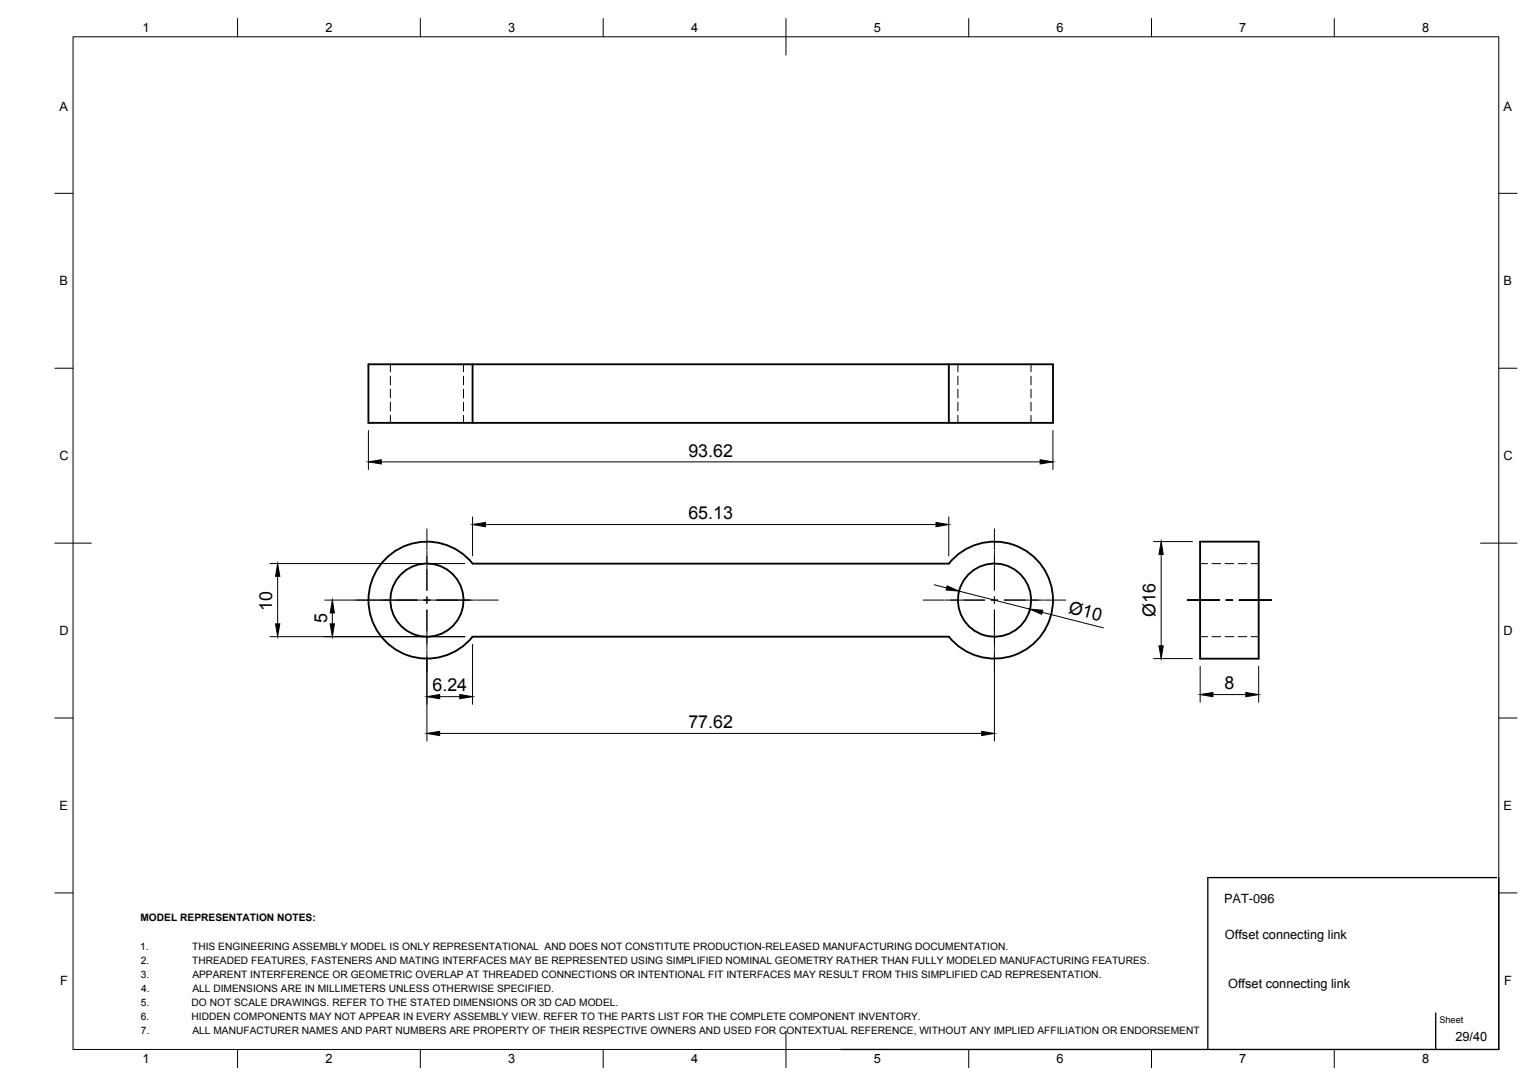
ISO-10303-21;
HEADER;
/* Generated by software containing ST-Developer
 * from STEP Tools, Inc. (www.steptools.com) 
 */

FILE_DESCRIPTION(
/* description */ ('PAT-096'),
/* implementation_level */ '2;1');

FILE_NAME(
/* name */ 'Offset connecting link.step',
/* time_stamp */ '2026-10-29T17:03:14-07:00',
/* author */ (''),
/* organization */ (''),
/* preprocessor_version */ 'ST-DEVELOPER v20.2',
/* originating_system */ 'Autodesk Translation Framework v15.17.0.0',
/* authorisation */ '');

FILE_SCHEMA (('AUTOMOTIVE_DESIGN { 1 0 10303 214 3 1 1 }'));
ENDSEC;

DATA;
#10=MECHANICAL_DESIGN_GEOMETRIC_PRESENTATION_REPRESENTATION('',(#426),#10650);
#356=SHAPE_REPRESENTATION_RELATIONSHIP('SRR','None',#10819,#387);
#387=ADVANCED_BREP_SHAPE_REPRESENTATION('',(#463),#10637);
#426=STYLED_ITEM('',(#11078),#463);
#463=MANIFOLD_SOLID_BREP('Body1',#5561);
#564=FACE_BOUND('',#1460,.T.);
#565=FACE_BOUND('',#1461,.T.);
#566=FACE_BOUND('',#1465,.T.);
#567=FACE_BOUND('',#1466,.T.);
#732=PLANE('',#6429);
#733=PLANE('',#6430);
#734=PLANE('',#6432);
#735=PLANE('',#6435);
#1028=FACE_OUTER_BOUND('',#1455,.T.);
#1029=FACE_OUTER_BOUND('',#1456,.T.);
#1030=FACE_OUTER_BOUND('',#1457,.T.);
#1031=FACE_OUTER_BOUND('',#1458,.T.);
#1032=FACE_OUTER_BOUND('',#1459,.T.);
#1033=FACE_OUTER_BOUND('',#1462,.T.);
#1034=FACE_OUTER_BOUND('',#1463,.T.);
#1035=FACE_OUTER_BOUND('',#1464,.T.);
#1455=EDGE_LOOP('',(#4695,#4696,#4697,#4698));
#1456=EDGE_LOOP('',(#4699,#4700,#4701,#4702));
#1457=EDGE_LOOP('',(#4703,#4704,#4705,#4706));
#1458=EDGE_LOOP('',(#4707,#4708,#4709,#4710));
#1459=EDGE_LOOP('',(#4711,#4712,#4713,#4714));
#1460=EDGE_LOOP('',(#4715));
#1461=EDGE_LOOP('',(#4716));
#1462=EDGE_LOOP('',(#4717,#4718,#4719,#4720));
#1463=EDGE_LOOP('',(#4721,#4722,#4723,#4724));
#1464=EDGE_LOOP('',(#4725,#4726,#4727,#4728));
#1465=EDGE_LOOP('',(#4729));
#1466=EDGE_LOOP('',(#4730));
#1824=LINE('',#10095,#2153);
#1825=LINE('',#10101,#2154);
#1826=LINE('',#10106,#2155);
#1827=LINE('',#10110,#2156);
#1828=LINE('',#10114,#2157);
#1829=LINE('',#10116,#2158);
#1830=LINE('',#10117,#2159);
#1831=LINE('',#10120,#2160);
#1832=LINE('',#10124,#2161);
#1833=LINE('',#10125,#2162);
#2153=VECTOR('',#7908,0.5);
#2154=VECTOR('',#7915,0.5);
#2155=VECTOR('',#7920,1.);
#2156=VECTOR('',#7923,1.);
#2157=VECTOR('',#7928,1.);
#2158=VECTOR('',#7929,1.);
#2159=VECTOR('',#7930,1.);
#2160=VECTOR('',#7933,1.);
#2161=VECTOR('',#7938,1.);
#2162=VECTOR('',#7939,1.);
#2495=CIRCLE('',#6421,0.5);
#2496=CIRCLE('',#6422,0.5);
#2497=CIRCLE('',#6424,0.5);
#2498=CIRCLE('',#6425,0.5);
#2499=CIRCLE('',#6427,0.800000000000001);
#2500=CIRCLE('',#6428,0.800000000000001);
#2501=CIRCLE('',#6431,0.8);
#2502=CIRCLE('',#6434,0.8);
#2911=VERTEX_POINT('',#10092);
#2912=VERTEX_POINT('',#10094);
#2913=VERTEX_POINT('',#10098);
#2914=VERTEX_POINT('',#10100);
#2915=VERTEX_POINT('',#10104);
#2916=VERTEX_POINT('',#10105);
#2917=VERTEX_POINT('',#10107);
#2918=VERTEX_POINT('',#10109);
#2919=VERTEX_POINT('',#10113);
#2920=VERTEX_POINT('',#10115);
#2921=VERTEX_POINT('',#10119);
#2922=VERTEX_POINT('',#10123);
#3526=EDGE_CURVE('',#2911,#2911,#2495,.T.);
#3527=EDGE_CURVE('',#2911,#2912,#1824,.T.);
#3528=EDGE_CURVE('',#2912,#2912,#2496,.T.);
#3529=EDGE_CURVE('',#2913,#2913,#2497,.T.);
#3530=EDGE_CURVE('',#2913,#2914,#1825,.T.);
#3531=EDGE_CURVE('',#2914,#2914,#2498,.T.);
#3532=EDGE_CURVE('',#2915,#2916,#1826,.T.);
#3533=EDGE_CURVE('',#2917,#2915,#2499,.T.);
#3534=EDGE_CURVE('',#2918,#2917,#1827,.T.);
#3535=EDGE_CURVE('',#2918,#2916,#2500,.T.);
#3536=EDGE_CURVE('',#2919,#2916,#1828,.T.);
#3537=EDGE_CURVE('',#2920,#2919,#1829,.T.);
#3538=EDGE_CURVE('',#2915,#2920,#1830,.T.);
#3539=EDGE_CURVE('',#2918,#2921,#1831,.T.);
#3540=EDGE_CURVE('',#2919,#2921,#2501,.T.);
#3541=EDGE_CURVE('',#2922,#2917,#1832,.T.);
#3542=EDGE_CURVE('',#2921,#2922,#1833,.T.);
#3543=EDGE_CURVE('',#2920,#2922,#2502,.T.);
#4695=ORIENTED_EDGE('',*,*,#3526,.F.);
#4696=ORIENTED_EDGE('',*,*,#3527,.T.);
#4697=ORIENTED_EDGE('',*,*,#3528,.F.);
#4698=ORIENTED_EDGE('',*,*,#3527,.F.);
#4699=ORIENTED_EDGE('',*,*,#3529,.F.);
#4700=ORIENTED_EDGE('',*,*,#3530,.T.);
#4701=ORIENTED_EDGE('',*,*,#3531,.F.);
#4702=ORIENTED_EDGE('',*,*,#3530,.F.);
#4703=ORIENTED_EDGE('',*,*,#3532,.F.);
#4704=ORIENTED_EDGE('',*,*,#3533,.F.);
#4705=ORIENTED_EDGE('',*,*,#3534,.F.);
#4706=ORIENTED_EDGE('',*,*,#3535,.T.);
#4707=ORIENTED_EDGE('',*,*,#3532,.T.);
#4708=ORIENTED_EDGE('',*,*,#3536,.F.);
#4709=ORIENTED_EDGE('',*,*,#3537,.F.);
#4710=ORIENTED_EDGE('',*,*,#3538,.F.);
#4711=ORIENTED_EDGE('',*,*,#3535,.F.);
#4712=ORIENTED_EDGE('',*,*,#3539,.T.);
#4713=ORIENTED_EDGE('',*,*,#3540,.F.);
#4714=ORIENTED_EDGE('',*,*,#3536,.T.);
#4715=ORIENTED_EDGE('',*,*,#3526,.T.);
#4716=ORIENTED_EDGE('',*,*,#3529,.T.);
#4717=ORIENTED_EDGE('',*,*,#3534,.T.);
#4718=ORIENTED_EDGE('',*,*,#3541,.F.);
#4719=ORIENTED_EDGE('',*,*,#3542,.F.);
#4720=ORIENTED_EDGE('',*,*,#3539,.F.);
#4721=ORIENTED_EDGE('',*,*,#3537,.T.);
#4722=ORIENTED_EDGE('',*,*,#3540,.T.);
#4723=ORIENTED_EDGE('',*,*,#3542,.T.);
#4724=ORIENTED_EDGE('',*,*,#3543,.F.);
#4725=ORIENTED_EDGE('',*,*,#3538,.T.);
#4726=ORIENTED_EDGE('',*,*,#3543,.T.);
#4727=ORIENTED_EDGE('',*,*,#3541,.T.);
#4728=ORIENTED_EDGE('',*,*,#3533,.T.);
#4729=ORIENTED_EDGE('',*,*,#3528,.T.);
#4730=ORIENTED_EDGE('',*,*,#3531,.T.);
#5158=CYLINDRICAL_SURFACE('',#6420,0.5);
#5159=CYLINDRICAL_SURFACE('',#6423,0.5);
#5160=CYLINDRICAL_SURFACE('',#6426,0.800000000000001);
#5161=CYLINDRICAL_SURFACE('',#6433,0.8);
#5433=ADVANCED_FACE('',(#1028),#5158,.F.);
#5434=ADVANCED_FACE('',(#1029),#5159,.F.);
#5435=ADVANCED_FACE('',(#1030),#5160,.T.);
#5436=ADVANCED_FACE('',(#1031),#732,.T.);
#5437=ADVANCED_FACE('',(#1032,#564,#565),#733,.F.);
#5438=ADVANCED_FACE('',(#1033),#734,.T.);
#5439=ADVANCED_FACE('',(#1034),#5161,.T.);
#5440=ADVANCED_FACE('',(#1035,#566,#567),#735,.T.);
#5561=CLOSED_SHELL('',(#5433,#5434,#5435,#5436,#5437,#5438,#5439,#5440));
#6419=AXIS2_PLACEMENT_3D('',#10090,#7902,#7903);
#6420=AXIS2_PLACEMENT_3D('',#10091,#7904,#7905);
#6421=AXIS2_PLACEMENT_3D('',#10093,#7906,#7907);
#6422=AXIS2_PLACEMENT_3D('',#10096,#7909,#7910);
#6423=AXIS2_PLACEMENT_3D('',#10097,#7911,#7912);
#6424=AXIS2_PLACEMENT_3D('',#10099,#7913,#7914);
#6425=AXIS2_PLACEMENT_3D('',#10102,#7916,#7917);
#6426=AXIS2_PLACEMENT_3D('',#10103,#7918,#7919);
#6427=AXIS2_PLACEMENT_3D('',#10108,#7921,#7922);
#6428=AXIS2_PLACEMENT_3D('',#10111,#7924,#7925);
#6429=AXIS2_PLACEMENT_3D('',#10112,#7926,#7927);
#6430=AXIS2_PLACEMENT_3D('',#10118,#7931,#7932);
#6431=AXIS2_PLACEMENT_3D('',#10121,#7934,#7935);
#6432=AXIS2_PLACEMENT_3D('',#10122,#7936,#7937);
#6433=AXIS2_PLACEMENT_3D('',#10126,#7940,#7941);
#6434=AXIS2_PLACEMENT_3D('',#10127,#7942,#7943);
#6435=AXIS2_PLACEMENT_3D('',#10128,#7944,#7945);
#7902=DIRECTION('axis',(0.,0.,1.));
#7903=DIRECTION('refdir',(1.,0.,0.));
#7904=DIRECTION('center_axis',(0.,0.,1.));
#7905=DIRECTION('ref_axis',(1.,0.,0.));
#7906=DIRECTION('center_axis',(0.,0.,1.));
#7907=DIRECTION('ref_axis',(1.,0.,0.));
#7908=DIRECTION('',(0.,0.,1.));
#7909=DIRECTION('center_axis',(0.,0.,-1.));
#7910=DIRECTION('ref_axis',(1.,0.,0.));
#7911=DIRECTION('center_axis',(0.,0.,1.));
#7912=DIRECTION('ref_axis',(1.,0.,0.));
#7913=DIRECTION('center_axis',(0.,0.,1.));
#7914=DIRECTION('ref_axis',(1.,0.,0.));
#7915=DIRECTION('',(0.,0.,1.));
#7916=DIRECTION('center_axis',(0.,0.,-1.));
#7917=DIRECTION('ref_axis',(1.,0.,0.));
#7918=DIRECTION('center_axis',(0.,0.,1.));
#7919=DIRECTION('ref_axis',(1.,0.,0.));
#7920=DIRECTION('',(0.,0.,-1.));
#7921=DIRECTION('center_axis',(0.,0.,1.));
#7922=DIRECTION('ref_axis',(1.,0.,0.));
#7923=DIRECTION('',(0.,0.,1.));
#7924=DIRECTION('center_axis',(0.,0.,1.));
#7925=DIRECTION('ref_axis',(1.,0.,0.));
#7926=DIRECTION('center_axis',(-0.257662650560332,0.966234939601246,0.));
#7927=DIRECTION('ref_axis',(-0.966234939601246,-0.257662650560332,0.));
#7928=DIRECTION('',(0.966234939601246,0.257662650560332,0.));
#7929=DIRECTION('',(0.,0.,-1.));
#7930=DIRECTION('',(-0.966234939601246,-0.257662650560332,0.));
#7931=DIRECTION('center_axis',(0.,0.,1.));
#7932=DIRECTION('ref_axis',(1.,0.,0.));
#7933=DIRECTION('',(-0.966234939601246,-0.257662650560332,0.));
#7934=DIRECTION('center_axis',(0.,0.,1.));
#7935=DIRECTION('ref_axis',(1.,0.,0.));
#7936=DIRECTION('center_axis',(0.257662650560332,-0.966234939601246,0.));
#7937=DIRECTION('ref_axis',(0.966234939601246,0.257662650560332,0.));
#7938=DIRECTION('',(0.966234939601246,0.257662650560332,0.));
#7939=DIRECTION('',(0.,0.,1.));
#7940=DIRECTION('center_axis',(0.,0.,1.));
#7941=DIRECTION('ref_axis',(-0.966234939601246,-0.257662650560332,0.));
#7942=DIRECTION('center_axis',(0.,0.,1.));
#7943=DIRECTION('ref_axis',(1.,0.,0.));
#7944=DIRECTION('center_axis',(0.,0.,1.));
#7945=DIRECTION('ref_axis',(1.,0.,0.));
#10090=CARTESIAN_POINT('',(0.,0.,0.));
#10091=CARTESIAN_POINT('Origin',(0.,2.,8.7));
#10092=CARTESIAN_POINT('',(-0.5,2.,8.8));
#10093=CARTESIAN_POINT('Origin',(0.,2.,8.8));
#10094=CARTESIAN_POINT('',(-0.5,2.,9.6));
#10095=CARTESIAN_POINT('',(-0.5,2.,8.7));
#10096=CARTESIAN_POINT('Origin',(0.,2.,9.6));
#10097=CARTESIAN_POINT('Origin',(7.5,4.,8.7));
#10098=CARTESIAN_POINT('',(7.,4.,8.8));
#10099=CARTESIAN_POINT('Origin',(7.5,4.,8.8));
#10100=CARTESIAN_POINT('',(7.,4.,9.6));
#10101=CARTESIAN_POINT('',(7.,4.,8.7));
#10102=CARTESIAN_POINT('Origin',(7.5,4.,9.6));
#10103=CARTESIAN_POINT('Origin',(7.5,4.,8.8));
#10104=CARTESIAN_POINT('',(6.7677551483406,4.32220719609949,9.6));
#10105=CARTESIAN_POINT('',(6.7677551483406,4.32220719609949,8.8));
#10106=CARTESIAN_POINT('',(6.7677551483406,4.32220719609949,8.8));
#10107=CARTESIAN_POINT('',(7.02541779890093,3.35597225649825,9.6));
#10108=CARTESIAN_POINT('Origin',(7.5,4.,9.6));
#10109=CARTESIAN_POINT('',(7.02541779890093,3.35597225649825,8.8));
#10110=CARTESIAN_POINT('',(7.02541779890093,3.35597225649825,8.8));
#10111=CARTESIAN_POINT('Origin',(7.5,4.,8.8));
#10112=CARTESIAN_POINT('Origin',(7.37116867471983,4.48311746980062,8.8));
#10113=CARTESIAN_POINT('',(0.474582201099072,2.64402774350175,8.8));
#10114=CARTESIAN_POINT('',(-0.128831325280166,2.48311746980062,8.8));
#10115=CARTESIAN_POINT('',(0.474582201099072,2.64402774350175,9.6));
#10116=CARTESIAN_POINT('',(0.474582201099072,2.64402774350175,8.8));
#10117=CARTESIAN_POINT('',(-0.128831325280166,2.48311746980062,9.6));
#10118=CARTESIAN_POINT('Origin',(0.,2.,8.8));
#10119=CARTESIAN_POINT('',(0.732244851659405,1.67779280390051,8.8));
#10120=CARTESIAN_POINT('',(7.62883132528017,3.51688253019938,8.8));
#10121=CARTESIAN_POINT('Origin',(0.,2.,8.8));
#10122=CARTESIAN_POINT('Origin',(0.128831325280166,1.51688253019938,8.8));
#10123=CARTESIAN_POINT('',(0.732244851659405,1.67779280390051,9.6));
#10124=CARTESIAN_POINT('',(7.62883132528017,3.51688253019938,9.6));
#10125=CARTESIAN_POINT('',(0.732244851659405,1.67779280390051,8.8));
#10126=CARTESIAN_POINT('Origin',(0.,2.,8.8));
#10127=CARTESIAN_POINT('Origin',(0.,2.,9.6));
#10128=CARTESIAN_POINT('Origin',(0.,2.,9.6));
#10598=UNCERTAINTY_MEASURE_WITH_UNIT(LENGTH_MEASURE(0.001),#10651,
'DISTANCE_ACCURACY_VALUE',
'Maximum model space distance between geometric entities at asserted c
onnectivities');
#10611=UNCERTAINTY_MEASURE_WITH_UNIT(LENGTH_MEASURE(0.001),#10651,
'DISTANCE_ACCURACY_VALUE',
'Maximum model space distance between geometric entities at asserted c
onnectivities');
#10637=(
GEOMETRIC_REPRESENTATION_CONTEXT(3)
GLOBAL_UNCERTAINTY_ASSIGNED_CONTEXT((#10598))
GLOBAL_UNIT_ASSIGNED_CONTEXT((#10651,#10653,#10654))
REPRESENTATION_CONTEXT('','3D')
);
#10650=(
GEOMETRIC_REPRESENTATION_CONTEXT(3)
GLOBAL_UNCERTAINTY_ASSIGNED_CONTEXT((#10611))
GLOBAL_UNIT_ASSIGNED_CONTEXT((#10651,#10653,#10654))
REPRESENTATION_CONTEXT('','3D')
);
#10651=(
LENGTH_UNIT()
NAMED_UNIT(*)
SI_UNIT(.CENTI.,.METRE.)
);
#10653=(
NAMED_UNIT(*)
PLANE_ANGLE_UNIT()
SI_UNIT($,.RADIAN.)
);
#10654=(
NAMED_UNIT(*)
SI_UNIT($,.STERADIAN.)
SOLID_ANGLE_UNIT()
);
#10680=SHAPE_DEFINITION_REPRESENTATION(#10723,#10819);
#10723=PRODUCT_DEFINITION_SHAPE('',$,#10858);
#10819=SHAPE_REPRESENTATION('',(#6419),#10637);
#10832=PRODUCT_DEFINITION_CONTEXT('part definition',#10948,'design');
#10858=PRODUCT_DEFINITION('Offset connecting link',
'Offset connecting link',#10896,#10832);
#10896=PRODUCT_DEFINITION_FORMATION('',$,#10975);
#10948=APPLICATION_CONTEXT(
'Core Data for Automotive Mechanical Design Process');
#10949=PRODUCT_CONTEXT('part definition',#10948,'mechanical');
#10975=PRODUCT('Offset connecting link','Offset connecting link',
'Offset connecting link',(#10949));
#11072=COLOUR_RGB('Off White',0.89,0.88,0.83);
#11073=FILL_AREA_STYLE_COLOUR('',#11072);
#11074=FILL_AREA_STYLE('',(#11073));
#11075=SURFACE_STYLE_FILL_AREA(#11074);
#11076=SURFACE_SIDE_STYLE('',(#11075));
#11077=SURFACE_STYLE_USAGE(.BOTH.,#11076);
#11078=PRESENTATION_STYLE_ASSIGNMENT((#11077));
ENDSEC;
END-ISO-10303-21;
